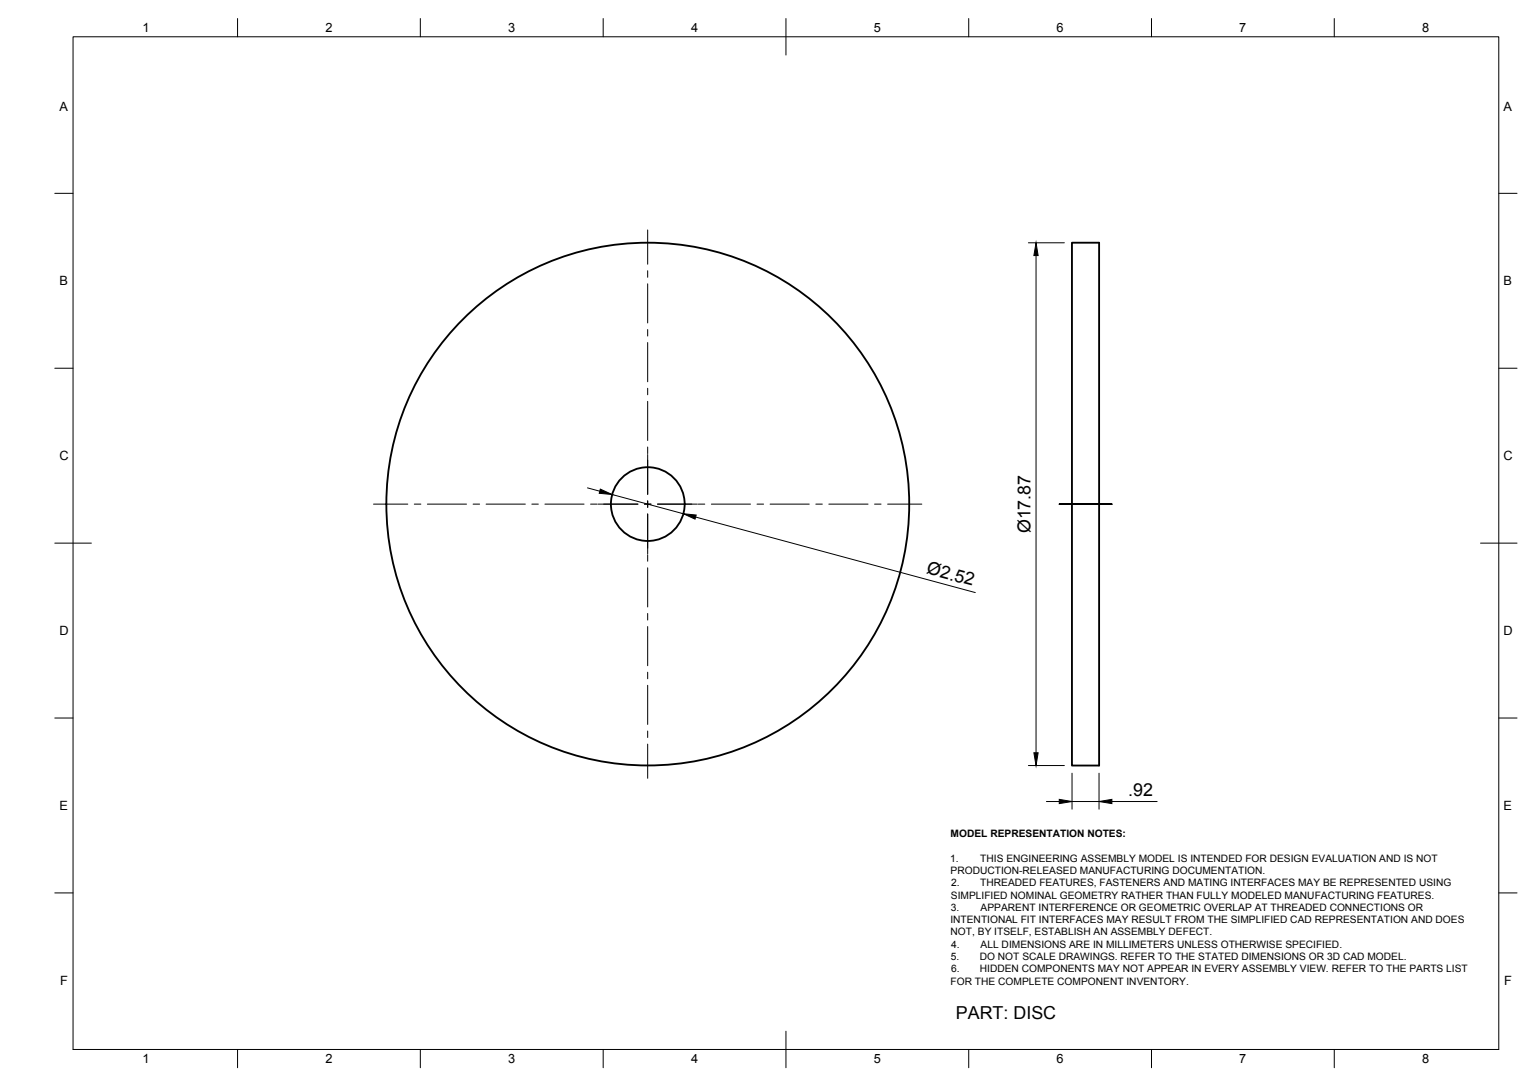
ISO-10303-21;
HEADER;
/* Generated by software containing ST-Developer
 * from STEP Tools, Inc. (www.steptools.com) 
 */

FILE_DESCRIPTION(
/* description */ (''),
/* implementation_level */ '2;1');

FILE_NAME(
/* name */ 'Disc.step',
/* time_stamp */ '2026-10-04T22:56:18-07:00',
/* author */ (''),
/* organization */ (''),
/* preprocessor_version */ 'ST-DEVELOPER v20.2',
/* originating_system */ 'Autodesk Translation Framework v15.15.0.0',
/* authorisation */ '');

FILE_SCHEMA (('AUTOMOTIVE_DESIGN { 1 0 10303 214 3 1 1 }'));
ENDSEC;

DATA;
#10=MECHANICAL_DESIGN_GEOMETRIC_PRESENTATION_REPRESENTATION('',(#193),#14544);
#177=SHAPE_REPRESENTATION_RELATIONSHIP('SRR','None',#14579,#185);
#185=ADVANCED_BREP_SHAPE_REPRESENTATION('',(#201),#14539);
#193=STYLED_ITEM('',(#14627),#201);
#201=MANIFOLD_SOLID_BREP('Body1',#1829);
#218=LINE('',#2701,#274);
#219=LINE('',#2706,#275);
#274=VECTOR('',#2270,8.93704988738917);
#275=VECTOR('',#2277,1.25945989284257);
#330=CYLINDRICAL_SURFACE('',#1986,8.93704988738917);
#331=CYLINDRICAL_SURFACE('',#1990,1.25945989284257);
#380=FACE_BOUND('',#542,.T.);
#381=FACE_BOUND('',#545,.T.);
#426=FACE_OUTER_BOUND('',#541,.T.);
#427=FACE_OUTER_BOUND('',#543,.T.);
#428=FACE_OUTER_BOUND('',#544,.T.);
#429=FACE_OUTER_BOUND('',#546,.T.);
#541=EDGE_LOOP('',(#1251));
#542=EDGE_LOOP('',(#1252));
#543=EDGE_LOOP('',(#1253,#1254,#1255,#1256));
#544=EDGE_LOOP('',(#1257));
#545=EDGE_LOOP('',(#1258));
#546=EDGE_LOOP('',(#1259,#1260,#1261,#1262));
#666=CIRCLE('',#1984,8.93704988738917);
#667=CIRCLE('',#1985,1.25945989284257);
#668=CIRCLE('',#1987,8.93704988738917);
#669=CIRCLE('',#1989,1.25945989284257);
#752=VERTEX_POINT('',#2694);
#753=VERTEX_POINT('',#2696);
#754=VERTEX_POINT('',#2699);
#755=VERTEX_POINT('',#2703);
#954=EDGE_CURVE('',#752,#752,#666,.T.);
#955=EDGE_CURVE('',#753,#753,#667,.T.);
#956=EDGE_CURVE('',#754,#754,#668,.T.);
#957=EDGE_CURVE('',#754,#752,#218,.T.);
#958=EDGE_CURVE('',#755,#755,#669,.T.);
#959=EDGE_CURVE('',#753,#755,#219,.T.);
#1251=ORIENTED_EDGE('',*,*,#954,.F.);
#1252=ORIENTED_EDGE('',*,*,#955,.F.);
#1253=ORIENTED_EDGE('',*,*,#956,.F.);
#1254=ORIENTED_EDGE('',*,*,#957,.T.);
#1255=ORIENTED_EDGE('',*,*,#954,.T.);
#1256=ORIENTED_EDGE('',*,*,#957,.F.);
#1257=ORIENTED_EDGE('',*,*,#956,.T.);
#1258=ORIENTED_EDGE('',*,*,#958,.F.);
#1259=ORIENTED_EDGE('',*,*,#955,.T.);
#1260=ORIENTED_EDGE('',*,*,#959,.T.);
#1261=ORIENTED_EDGE('',*,*,#958,.T.);
#1262=ORIENTED_EDGE('',*,*,#959,.F.);
#1697=PLANE('',#1983);
#1698=PLANE('',#1988);
#1748=ADVANCED_FACE('',(#426,#380),#1697,.F.);
#1749=ADVANCED_FACE('',(#427),#330,.T.);
#1750=ADVANCED_FACE('',(#428,#381),#1698,.T.);
#1751=ADVANCED_FACE('',(#429),#331,.F.);
#1829=CLOSED_SHELL('',(#1748,#1749,#1750,#1751));
#1982=AXIS2_PLACEMENT_3D('',#2692,#2258,#2259);
#1983=AXIS2_PLACEMENT_3D('',#2693,#2260,#2261);
#1984=AXIS2_PLACEMENT_3D('',#2695,#2262,#2263);
#1985=AXIS2_PLACEMENT_3D('',#2697,#2264,#2265);
#1986=AXIS2_PLACEMENT_3D('',#2698,#2266,#2267);
#1987=AXIS2_PLACEMENT_3D('',#2700,#2268,#2269);
#1988=AXIS2_PLACEMENT_3D('',#2702,#2271,#2272);
#1989=AXIS2_PLACEMENT_3D('',#2704,#2273,#2274);
#1990=AXIS2_PLACEMENT_3D('',#2705,#2275,#2276);
#2258=DIRECTION('axis',(0.,0.,1.));
#2259=DIRECTION('refdir',(1.,0.,0.));
#2260=DIRECTION('center_axis',(0.,0.,1.));
#2261=DIRECTION('ref_axis',(1.,0.,0.));
#2262=DIRECTION('center_axis',(0.,0.,1.));
#2263=DIRECTION('ref_axis',(1.,0.,0.));
#2264=DIRECTION('center_axis',(0.,0.,-1.));
#2265=DIRECTION('ref_axis',(1.,0.,0.));
#2266=DIRECTION('center_axis',(0.,0.,1.));
#2267=DIRECTION('ref_axis',(1.,0.,0.));
#2268=DIRECTION('center_axis',(0.,0.,1.));
#2269=DIRECTION('ref_axis',(1.,0.,0.));
#2270=DIRECTION('',(0.,0.,-1.));
#2271=DIRECTION('center_axis',(0.,0.,1.));
#2272=DIRECTION('ref_axis',(1.,0.,0.));
#2273=DIRECTION('center_axis',(0.,0.,1.));
#2274=DIRECTION('ref_axis',(1.,0.,0.));
#2275=DIRECTION('center_axis',(0.,0.,1.));
#2276=DIRECTION('ref_axis',(1.,0.,0.));
#2277=DIRECTION('',(0.,0.,1.));
#2692=CARTESIAN_POINT('',(0.,0.,0.));
#2693=CARTESIAN_POINT('Origin',(0.,0.,61.3445102174369));
#2694=CARTESIAN_POINT('',(-8.93704988738917,-1.09447295384114E-15,61.3445102174369));
#2695=CARTESIAN_POINT('Origin',(0.,0.,61.3445102174369));
#2696=CARTESIAN_POINT('',(-1.25945989284257,1.54239352642412E-16,61.3445102174369));
#2697=CARTESIAN_POINT('Origin',(0.,0.,61.3445102174369));
#2698=CARTESIAN_POINT('Origin',(0.,0.,61.8066396156573));
#2699=CARTESIAN_POINT('',(-8.93704988738917,-1.09447295384114E-15,62.2687690138778));
#2700=CARTESIAN_POINT('Origin',(0.,0.,62.2687690138778));
#2701=CARTESIAN_POINT('',(-8.93704988738917,-1.09447295384114E-15,61.8066396156573));
#2702=CARTESIAN_POINT('Origin',(1.25945989284257,0.,62.2687690138778));
#2703=CARTESIAN_POINT('',(-1.25945989284257,-1.54239352642412E-16,62.2687690138778));
#2704=CARTESIAN_POINT('Origin',(0.,0.,62.2687690138778));
#2705=CARTESIAN_POINT('Origin',(0.,0.,60.205945294667));
#2706=CARTESIAN_POINT('',(-1.25945989284257,-1.54239352642412E-16,60.205945294667));
#14529=UNCERTAINTY_MEASURE_WITH_UNIT(LENGTH_MEASURE(0.01),#14545,
'DISTANCE_ACCURACY_VALUE',
'Maximum model space distance between geometric entities at asserted c
onnectivities');
#14534=UNCERTAINTY_MEASURE_WITH_UNIT(LENGTH_MEASURE(0.01),#14545,
'DISTANCE_ACCURACY_VALUE',
'Maximum model space distance between geometric entities at asserted c
onnectivities');
#14539=(
GEOMETRIC_REPRESENTATION_CONTEXT(3)
GLOBAL_UNCERTAINTY_ASSIGNED_CONTEXT((#14529))
GLOBAL_UNIT_ASSIGNED_CONTEXT((#14545,#14547,#14548))
REPRESENTATION_CONTEXT('','3D')
);
#14544=(
GEOMETRIC_REPRESENTATION_CONTEXT(3)
GLOBAL_UNCERTAINTY_ASSIGNED_CONTEXT((#14534))
GLOBAL_UNIT_ASSIGNED_CONTEXT((#14545,#14547,#14548))
REPRESENTATION_CONTEXT('','3D')
);
#14545=(
LENGTH_UNIT()
NAMED_UNIT(*)
SI_UNIT(.MILLI.,.METRE.)
);
#14547=(
NAMED_UNIT(*)
PLANE_ANGLE_UNIT()
SI_UNIT($,.RADIAN.)
);
#14548=(
NAMED_UNIT(*)
SI_UNIT($,.STERADIAN.)
SOLID_ANGLE_UNIT()
);
#14553=SHAPE_DEFINITION_REPRESENTATION(#14562,#14579);
#14562=PRODUCT_DEFINITION_SHAPE('',$,#14589);
#14579=SHAPE_REPRESENTATION('',(#1982),#14539);
#14584=PRODUCT_DEFINITION_CONTEXT('part definition',#14613,'design');
#14589=PRODUCT_DEFINITION('Disc','Disc',#14598,#14584);
#14598=PRODUCT_DEFINITION_FORMATION('',$,#14619);
#14613=APPLICATION_CONTEXT(
'Core Data for Automotive Mechanical Design Process');
#14614=PRODUCT_CONTEXT('part definition',#14613,'mechanical');
#14619=PRODUCT('Disc','Disc',$,(#14614));
#14627=PRESENTATION_STYLE_ASSIGNMENT((#14631));
#14631=SURFACE_STYLE_USAGE(.BOTH.,#14635);
#14635=SURFACE_SIDE_STYLE('',(#14639));
#14639=SURFACE_STYLE_FILL_AREA(#14643);
#14643=FILL_AREA_STYLE('Opaque(203,203,203)',(#14647));
#14647=FILL_AREA_STYLE_COLOUR('Opaque(203,203,203)',#14651);
#14651=COLOUR_RGB('Opaque(203,203,203)', 0.31764706, 0.68627451, 0.89019608);
ENDSEC;
END-ISO-10303-21;
